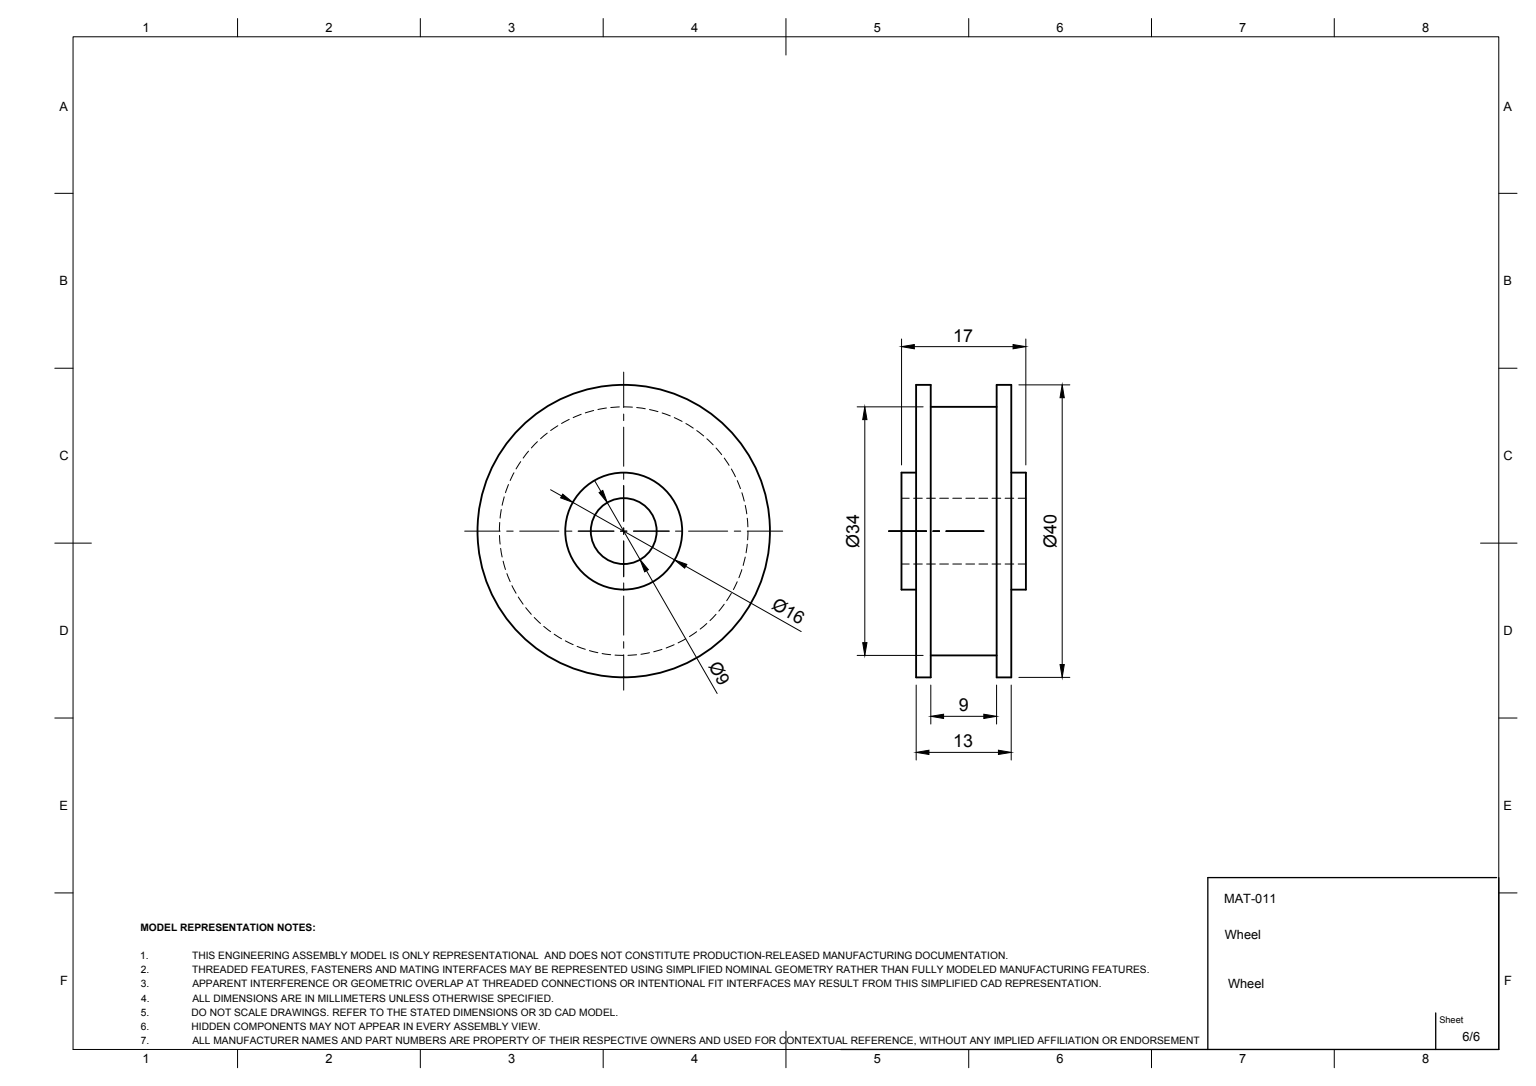
ISO-10303-21;
HEADER;
/* Generated by software containing ST-Developer
 * from STEP Tools, Inc. (www.steptools.com) 
 */

FILE_DESCRIPTION(
/* description */ ('STEP AP214'),
/* implementation_level */ '2;1');

FILE_NAME(
/* name */ 'Wheel.step',
/* time_stamp */ '2026-11-14T05:56:09-08:00',
/* author */ (''),
/* organization */ (''),
/* preprocessor_version */ 'ST-DEVELOPER v20.2',
/* originating_system */ 'Autodesk Translation Framework v15.17.0.0',
/* authorisation */ '');

FILE_SCHEMA (('AUTOMOTIVE_DESIGN { 1 0 10303 214 3 1 1 }'));
ENDSEC;

DATA;
#10=MECHANICAL_DESIGN_GEOMETRIC_PRESENTATION_REPRESENTATION('',(#106),#3207);
#94=SHAPE_REPRESENTATION_RELATIONSHIP('SRR','None',#3246,#100);
#100=ADVANCED_BREP_SHAPE_REPRESENTATION('',(#112),#3205);
#106=STYLED_ITEM('',(#3282),#112);
#112=MANIFOLD_SOLID_BREP('Body1',#1284);
#138=PLANE('',#1459);
#139=PLANE('',#1460);
#140=PLANE('',#1461);
#141=PLANE('',#1462);
#142=PLANE('',#1463);
#143=PLANE('',#1464);
#202=LINE('',#2162,#269);
#203=LINE('',#2168,#270);
#204=LINE('',#2174,#271);
#205=LINE('',#2180,#272);
#206=LINE('',#2186,#273);
#207=LINE('',#2192,#274);
#269=VECTOR('',#1748,8.);
#270=VECTOR('',#1755,20.);
#271=VECTOR('',#1762,17.);
#272=VECTOR('',#1769,20.);
#273=VECTOR('',#1776,8.);
#274=VECTOR('',#1783,4.5);
#299=CYLINDRICAL_SURFACE('',#1441,8.);
#300=CYLINDRICAL_SURFACE('',#1444,20.);
#301=CYLINDRICAL_SURFACE('',#1447,17.);
#302=CYLINDRICAL_SURFACE('',#1450,20.);
#303=CYLINDRICAL_SURFACE('',#1453,8.);
#304=CYLINDRICAL_SURFACE('',#1456,4.5);
#320=FACE_BOUND('',#482,.T.);
#321=FACE_BOUND('',#484,.T.);
#322=FACE_BOUND('',#486,.T.);
#323=FACE_BOUND('',#488,.T.);
#324=FACE_BOUND('',#490,.T.);
#325=FACE_BOUND('',#492,.T.);
#388=FACE_OUTER_BOUND('',#475,.T.);
#389=FACE_OUTER_BOUND('',#476,.T.);
#390=FACE_OUTER_BOUND('',#477,.T.);
#391=FACE_OUTER_BOUND('',#478,.T.);
#392=FACE_OUTER_BOUND('',#479,.T.);
#393=FACE_OUTER_BOUND('',#480,.T.);
#394=FACE_OUTER_BOUND('',#481,.T.);
#395=FACE_OUTER_BOUND('',#483,.T.);
#396=FACE_OUTER_BOUND('',#485,.T.);
#397=FACE_OUTER_BOUND('',#487,.T.);
#398=FACE_OUTER_BOUND('',#489,.T.);
#399=FACE_OUTER_BOUND('',#491,.T.);
#475=EDGE_LOOP('',(#1045,#1046,#1047,#1048));
#476=EDGE_LOOP('',(#1049,#1050,#1051,#1052));
#477=EDGE_LOOP('',(#1053,#1054,#1055,#1056));
#478=EDGE_LOOP('',(#1057,#1058,#1059,#1060));
#479=EDGE_LOOP('',(#1061,#1062,#1063,#1064));
#480=EDGE_LOOP('',(#1065,#1066,#1067,#1068));
#481=EDGE_LOOP('',(#1069));
#482=EDGE_LOOP('',(#1070));
#483=EDGE_LOOP('',(#1071));
#484=EDGE_LOOP('',(#1072));
#485=EDGE_LOOP('',(#1073));
#486=EDGE_LOOP('',(#1074));
#487=EDGE_LOOP('',(#1075));
#488=EDGE_LOOP('',(#1076));
#489=EDGE_LOOP('',(#1077));
#490=EDGE_LOOP('',(#1078));
#491=EDGE_LOOP('',(#1079));
#492=EDGE_LOOP('',(#1080));
#557=CIRCLE('',#1442,8.);
#558=CIRCLE('',#1443,8.);
#559=CIRCLE('',#1445,20.);
#560=CIRCLE('',#1446,20.);
#561=CIRCLE('',#1448,17.);
#562=CIRCLE('',#1449,17.);
#563=CIRCLE('',#1451,20.);
#564=CIRCLE('',#1452,20.);
#565=CIRCLE('',#1454,8.);
#566=CIRCLE('',#1455,8.);
#567=CIRCLE('',#1457,4.5);
#568=CIRCLE('',#1458,4.5);
#645=VERTEX_POINT('',#2159);
#646=VERTEX_POINT('',#2161);
#647=VERTEX_POINT('',#2165);
#648=VERTEX_POINT('',#2167);
#649=VERTEX_POINT('',#2171);
#650=VERTEX_POINT('',#2173);
#651=VERTEX_POINT('',#2177);
#652=VERTEX_POINT('',#2179);
#653=VERTEX_POINT('',#2183);
#654=VERTEX_POINT('',#2185);
#655=VERTEX_POINT('',#2189);
#656=VERTEX_POINT('',#2191);
#786=EDGE_CURVE('',#645,#645,#557,.T.);
#787=EDGE_CURVE('',#645,#646,#202,.T.);
#788=EDGE_CURVE('',#646,#646,#558,.T.);
#789=EDGE_CURVE('',#647,#647,#559,.T.);
#790=EDGE_CURVE('',#647,#648,#203,.T.);
#791=EDGE_CURVE('',#648,#648,#560,.T.);
#792=EDGE_CURVE('',#649,#649,#561,.T.);
#793=EDGE_CURVE('',#649,#650,#204,.T.);
#794=EDGE_CURVE('',#650,#650,#562,.T.);
#795=EDGE_CURVE('',#651,#651,#563,.T.);
#796=EDGE_CURVE('',#651,#652,#205,.T.);
#797=EDGE_CURVE('',#652,#652,#564,.T.);
#798=EDGE_CURVE('',#653,#653,#565,.T.);
#799=EDGE_CURVE('',#653,#654,#206,.T.);
#800=EDGE_CURVE('',#654,#654,#566,.T.);
#801=EDGE_CURVE('',#655,#655,#567,.T.);
#802=EDGE_CURVE('',#655,#656,#207,.T.);
#803=EDGE_CURVE('',#656,#656,#568,.T.);
#1045=ORIENTED_EDGE('',*,*,#786,.F.);
#1046=ORIENTED_EDGE('',*,*,#787,.T.);
#1047=ORIENTED_EDGE('',*,*,#788,.T.);
#1048=ORIENTED_EDGE('',*,*,#787,.F.);
#1049=ORIENTED_EDGE('',*,*,#789,.F.);
#1050=ORIENTED_EDGE('',*,*,#790,.T.);
#1051=ORIENTED_EDGE('',*,*,#791,.T.);
#1052=ORIENTED_EDGE('',*,*,#790,.F.);
#1053=ORIENTED_EDGE('',*,*,#792,.F.);
#1054=ORIENTED_EDGE('',*,*,#793,.T.);
#1055=ORIENTED_EDGE('',*,*,#794,.T.);
#1056=ORIENTED_EDGE('',*,*,#793,.F.);
#1057=ORIENTED_EDGE('',*,*,#795,.F.);
#1058=ORIENTED_EDGE('',*,*,#796,.T.);
#1059=ORIENTED_EDGE('',*,*,#797,.T.);
#1060=ORIENTED_EDGE('',*,*,#796,.F.);
#1061=ORIENTED_EDGE('',*,*,#798,.F.);
#1062=ORIENTED_EDGE('',*,*,#799,.T.);
#1063=ORIENTED_EDGE('',*,*,#800,.T.);
#1064=ORIENTED_EDGE('',*,*,#799,.F.);
#1065=ORIENTED_EDGE('',*,*,#801,.F.);
#1066=ORIENTED_EDGE('',*,*,#802,.T.);
#1067=ORIENTED_EDGE('',*,*,#803,.T.);
#1068=ORIENTED_EDGE('',*,*,#802,.F.);
#1069=ORIENTED_EDGE('',*,*,#798,.T.);
#1070=ORIENTED_EDGE('',*,*,#803,.F.);
#1071=ORIENTED_EDGE('',*,*,#795,.T.);
#1072=ORIENTED_EDGE('',*,*,#800,.F.);
#1073=ORIENTED_EDGE('',*,*,#797,.F.);
#1074=ORIENTED_EDGE('',*,*,#792,.T.);
#1075=ORIENTED_EDGE('',*,*,#789,.T.);
#1076=ORIENTED_EDGE('',*,*,#794,.F.);
#1077=ORIENTED_EDGE('',*,*,#791,.F.);
#1078=ORIENTED_EDGE('',*,*,#786,.T.);
#1079=ORIENTED_EDGE('',*,*,#788,.F.);
#1080=ORIENTED_EDGE('',*,*,#801,.T.);
#1246=ADVANCED_FACE('',(#388),#299,.T.);
#1247=ADVANCED_FACE('',(#389),#300,.T.);
#1248=ADVANCED_FACE('',(#390),#301,.T.);
#1249=ADVANCED_FACE('',(#391),#302,.T.);
#1250=ADVANCED_FACE('',(#392),#303,.T.);
#1251=ADVANCED_FACE('',(#393),#304,.F.);
#1252=ADVANCED_FACE('',(#394,#320),#138,.T.);
#1253=ADVANCED_FACE('',(#395,#321),#139,.T.);
#1254=ADVANCED_FACE('',(#396,#322),#140,.T.);
#1255=ADVANCED_FACE('',(#397,#323),#141,.F.);
#1256=ADVANCED_FACE('',(#398,#324),#142,.F.);
#1257=ADVANCED_FACE('',(#399,#325),#143,.F.);
#1284=CLOSED_SHELL('',(#1246,#1247,#1248,#1249,#1250,#1251,#1252,#1253,
#1254,#1255,#1256,#1257));
#1440=AXIS2_PLACEMENT_3D('',#2157,#1742,#1743);
#1441=AXIS2_PLACEMENT_3D('',#2158,#1744,#1745);
#1442=AXIS2_PLACEMENT_3D('',#2160,#1746,#1747);
#1443=AXIS2_PLACEMENT_3D('',#2163,#1749,#1750);
#1444=AXIS2_PLACEMENT_3D('',#2164,#1751,#1752);
#1445=AXIS2_PLACEMENT_3D('',#2166,#1753,#1754);
#1446=AXIS2_PLACEMENT_3D('',#2169,#1756,#1757);
#1447=AXIS2_PLACEMENT_3D('',#2170,#1758,#1759);
#1448=AXIS2_PLACEMENT_3D('',#2172,#1760,#1761);
#1449=AXIS2_PLACEMENT_3D('',#2175,#1763,#1764);
#1450=AXIS2_PLACEMENT_3D('',#2176,#1765,#1766);
#1451=AXIS2_PLACEMENT_3D('',#2178,#1767,#1768);
#1452=AXIS2_PLACEMENT_3D('',#2181,#1770,#1771);
#1453=AXIS2_PLACEMENT_3D('',#2182,#1772,#1773);
#1454=AXIS2_PLACEMENT_3D('',#2184,#1774,#1775);
#1455=AXIS2_PLACEMENT_3D('',#2187,#1777,#1778);
#1456=AXIS2_PLACEMENT_3D('',#2188,#1779,#1780);
#1457=AXIS2_PLACEMENT_3D('',#2190,#1781,#1782);
#1458=AXIS2_PLACEMENT_3D('',#2193,#1784,#1785);
#1459=AXIS2_PLACEMENT_3D('',#2194,#1786,#1787);
#1460=AXIS2_PLACEMENT_3D('',#2195,#1788,#1789);
#1461=AXIS2_PLACEMENT_3D('',#2196,#1790,#1791);
#1462=AXIS2_PLACEMENT_3D('',#2197,#1792,#1793);
#1463=AXIS2_PLACEMENT_3D('',#2198,#1794,#1795);
#1464=AXIS2_PLACEMENT_3D('',#2199,#1796,#1797);
#1742=DIRECTION('axis',(0.,0.,1.));
#1743=DIRECTION('refdir',(1.,0.,0.));
#1744=DIRECTION('center_axis',(1.,0.,0.));
#1745=DIRECTION('ref_axis',(0.,0.,-1.));
#1746=DIRECTION('center_axis',(1.,0.,0.));
#1747=DIRECTION('ref_axis',(0.,0.,-1.));
#1748=DIRECTION('',(-1.,0.,0.));
#1749=DIRECTION('center_axis',(1.,0.,0.));
#1750=DIRECTION('ref_axis',(0.,0.,-1.));
#1751=DIRECTION('center_axis',(1.,0.,0.));
#1752=DIRECTION('ref_axis',(0.,0.,-1.));
#1753=DIRECTION('center_axis',(1.,0.,0.));
#1754=DIRECTION('ref_axis',(0.,0.,-1.));
#1755=DIRECTION('',(-1.,0.,0.));
#1756=DIRECTION('center_axis',(1.,0.,0.));
#1757=DIRECTION('ref_axis',(0.,0.,-1.));
#1758=DIRECTION('center_axis',(1.,0.,0.));
#1759=DIRECTION('ref_axis',(0.,0.,-1.));
#1760=DIRECTION('center_axis',(1.,0.,0.));
#1761=DIRECTION('ref_axis',(0.,0.,-1.));
#1762=DIRECTION('',(-1.,0.,0.));
#1763=DIRECTION('center_axis',(1.,0.,0.));
#1764=DIRECTION('ref_axis',(0.,0.,-1.));
#1765=DIRECTION('center_axis',(1.,0.,0.));
#1766=DIRECTION('ref_axis',(0.,0.,-1.));
#1767=DIRECTION('center_axis',(1.,0.,0.));
#1768=DIRECTION('ref_axis',(0.,0.,-1.));
#1769=DIRECTION('',(-1.,0.,0.));
#1770=DIRECTION('center_axis',(1.,0.,0.));
#1771=DIRECTION('ref_axis',(0.,0.,-1.));
#1772=DIRECTION('center_axis',(1.,0.,0.));
#1773=DIRECTION('ref_axis',(0.,0.,-1.));
#1774=DIRECTION('center_axis',(1.,0.,0.));
#1775=DIRECTION('ref_axis',(0.,0.,-1.));
#1776=DIRECTION('',(-1.,0.,0.));
#1777=DIRECTION('center_axis',(1.,0.,0.));
#1778=DIRECTION('ref_axis',(0.,0.,-1.));
#1779=DIRECTION('center_axis',(1.,0.,0.));
#1780=DIRECTION('ref_axis',(0.,0.,-1.));
#1781=DIRECTION('center_axis',(1.,0.,0.));
#1782=DIRECTION('ref_axis',(0.,0.,-1.));
#1783=DIRECTION('',(1.,0.,0.));
#1784=DIRECTION('center_axis',(1.,0.,0.));
#1785=DIRECTION('ref_axis',(0.,0.,-1.));
#1786=DIRECTION('center_axis',(1.,0.,0.));
#1787=DIRECTION('ref_axis',(0.,0.,-1.));
#1788=DIRECTION('center_axis',(1.,0.,0.));
#1789=DIRECTION('ref_axis',(0.,0.,-1.));
#1790=DIRECTION('center_axis',(-1.,0.,0.));
#1791=DIRECTION('ref_axis',(0.,0.,1.));
#1792=DIRECTION('center_axis',(-1.,0.,0.));
#1793=DIRECTION('ref_axis',(0.,0.,1.));
#1794=DIRECTION('center_axis',(1.,0.,0.));
#1795=DIRECTION('ref_axis',(0.,0.,-1.));
#1796=DIRECTION('center_axis',(1.,0.,0.));
#1797=DIRECTION('ref_axis',(0.,0.,-1.));
#2157=CARTESIAN_POINT('',(0.,0.,0.));
#2158=CARTESIAN_POINT('Origin',(-8.50000000000001,0.,0.));
#2159=CARTESIAN_POINT('',(-6.50000000000001,-9.79717439317883E-16,8.));
#2160=CARTESIAN_POINT('Origin',(-6.50000000000001,0.,0.));
#2161=CARTESIAN_POINT('',(-8.50000000000001,-9.79717439317883E-16,8.));
#2162=CARTESIAN_POINT('',(-8.50000000000001,-9.79717439317883E-16,8.));
#2163=CARTESIAN_POINT('Origin',(-8.50000000000001,0.,0.));
#2164=CARTESIAN_POINT('Origin',(-8.50000000000001,0.,0.));
#2165=CARTESIAN_POINT('',(-4.50000000000001,-2.44929359829471E-15,20.));
#2166=CARTESIAN_POINT('Origin',(-4.50000000000001,0.,0.));
#2167=CARTESIAN_POINT('',(-6.50000000000001,-2.44929359829471E-15,20.));
#2168=CARTESIAN_POINT('',(-8.50000000000001,-2.44929359829471E-15,20.));
#2169=CARTESIAN_POINT('Origin',(-6.50000000000001,0.,0.));
#2170=CARTESIAN_POINT('Origin',(-8.50000000000001,0.,0.));
#2171=CARTESIAN_POINT('',(4.50000000000001,-2.0818995585505E-15,17.));
#2172=CARTESIAN_POINT('Origin',(4.50000000000001,0.,0.));
#2173=CARTESIAN_POINT('',(-4.50000000000001,-2.0818995585505E-15,17.));
#2174=CARTESIAN_POINT('',(-8.50000000000001,-2.0818995585505E-15,17.));
#2175=CARTESIAN_POINT('Origin',(-4.50000000000001,0.,0.));
#2176=CARTESIAN_POINT('Origin',(-8.50000000000001,0.,0.));
#2177=CARTESIAN_POINT('',(6.50000000000001,-2.44929359829471E-15,20.));
#2178=CARTESIAN_POINT('Origin',(6.50000000000001,0.,0.));
#2179=CARTESIAN_POINT('',(4.50000000000001,-2.44929359829471E-15,20.));
#2180=CARTESIAN_POINT('',(-8.50000000000001,-2.44929359829471E-15,20.));
#2181=CARTESIAN_POINT('Origin',(4.50000000000001,0.,0.));
#2182=CARTESIAN_POINT('Origin',(-8.50000000000001,0.,0.));
#2183=CARTESIAN_POINT('',(8.50000000000001,-9.79717439317883E-16,8.));
#2184=CARTESIAN_POINT('Origin',(8.50000000000001,0.,0.));
#2185=CARTESIAN_POINT('',(6.50000000000001,-9.79717439317883E-16,8.));
#2186=CARTESIAN_POINT('',(-8.50000000000001,-9.79717439317883E-16,8.));
#2187=CARTESIAN_POINT('Origin',(6.50000000000001,0.,0.));
#2188=CARTESIAN_POINT('Origin',(-8.50000000000001,0.,0.));
#2189=CARTESIAN_POINT('',(-8.50000000000001,-5.51091059616309E-16,4.5));
#2190=CARTESIAN_POINT('Origin',(-8.50000000000001,0.,0.));
#2191=CARTESIAN_POINT('',(8.50000000000001,-5.51091059616309E-16,4.5));
#2192=CARTESIAN_POINT('',(-8.50000000000001,-5.51091059616309E-16,4.5));
#2193=CARTESIAN_POINT('Origin',(8.50000000000001,0.,0.));
#2194=CARTESIAN_POINT('Origin',(8.50000000000001,0.,0.));
#2195=CARTESIAN_POINT('Origin',(6.50000000000001,0.,0.));
#2196=CARTESIAN_POINT('Origin',(4.50000000000001,0.,0.));
#2197=CARTESIAN_POINT('Origin',(-4.50000000000001,0.,0.));
#2198=CARTESIAN_POINT('Origin',(-6.50000000000001,0.,0.));
#2199=CARTESIAN_POINT('Origin',(-8.50000000000001,0.,0.));
#3197=UNCERTAINTY_MEASURE_WITH_UNIT(LENGTH_MEASURE(0.01),#3208,
'DISTANCE_ACCURACY_VALUE',
'Maximum model space distance between geometric entities at asserted c
onnectivities');
#3199=UNCERTAINTY_MEASURE_WITH_UNIT(LENGTH_MEASURE(0.01),#3208,
'DISTANCE_ACCURACY_VALUE',
'Maximum model space distance between geometric entities at asserted c
onnectivities');
#3205=(
GEOMETRIC_REPRESENTATION_CONTEXT(3)
GLOBAL_UNCERTAINTY_ASSIGNED_CONTEXT((#3197))
GLOBAL_UNIT_ASSIGNED_CONTEXT((#3208,#3210,#3211))
REPRESENTATION_CONTEXT('','3D')
);
#3207=(
GEOMETRIC_REPRESENTATION_CONTEXT(3)
GLOBAL_UNCERTAINTY_ASSIGNED_CONTEXT((#3199))
GLOBAL_UNIT_ASSIGNED_CONTEXT((#3208,#3210,#3211))
REPRESENTATION_CONTEXT('','3D')
);
#3208=(
LENGTH_UNIT()
NAMED_UNIT(*)
SI_UNIT(.MILLI.,.METRE.)
);
#3210=(
NAMED_UNIT(*)
PLANE_ANGLE_UNIT()
SI_UNIT($,.RADIAN.)
);
#3211=(
NAMED_UNIT(*)
SI_UNIT($,.STERADIAN.)
SOLID_ANGLE_UNIT()
);
#3217=SHAPE_DEFINITION_REPRESENTATION(#3224,#3246);
#3224=PRODUCT_DEFINITION_SHAPE('',$,#3254);
#3246=SHAPE_REPRESENTATION('',(#1440),#3205);
#3248=PRODUCT_DEFINITION_CONTEXT('part definition',#3271,'design');
#3254=PRODUCT_DEFINITION('Wheel','Wheel',#3261,#3248);
#3261=PRODUCT_DEFINITION_FORMATION('',$,#3278);
#3271=APPLICATION_CONTEXT(
'Core Data for Automotive Mechanical Design Process');
#3272=PRODUCT_CONTEXT('part definition',#3271,'mechanical');
#3278=PRODUCT('Wheel','Wheel','Wheel',(#3272));
#3282=PRESENTATION_STYLE_ASSIGNMENT((#3286));
#3286=SURFACE_STYLE_USAGE(.BOTH.,#3290);
#3290=SURFACE_SIDE_STYLE('',(#3294));
#3294=SURFACE_STYLE_FILL_AREA(#3298);
#3298=FILL_AREA_STYLE('Opaque(227,224,212)',(#3302));
#3302=FILL_AREA_STYLE_COLOUR('Opaque(227,224,212)',#3306);
#3306=COLOUR_RGB('Opaque(227,224,212)',0.890196078431372,0.87843137254902,
0.831372549019608);
ENDSEC;
END-ISO-10303-21;
